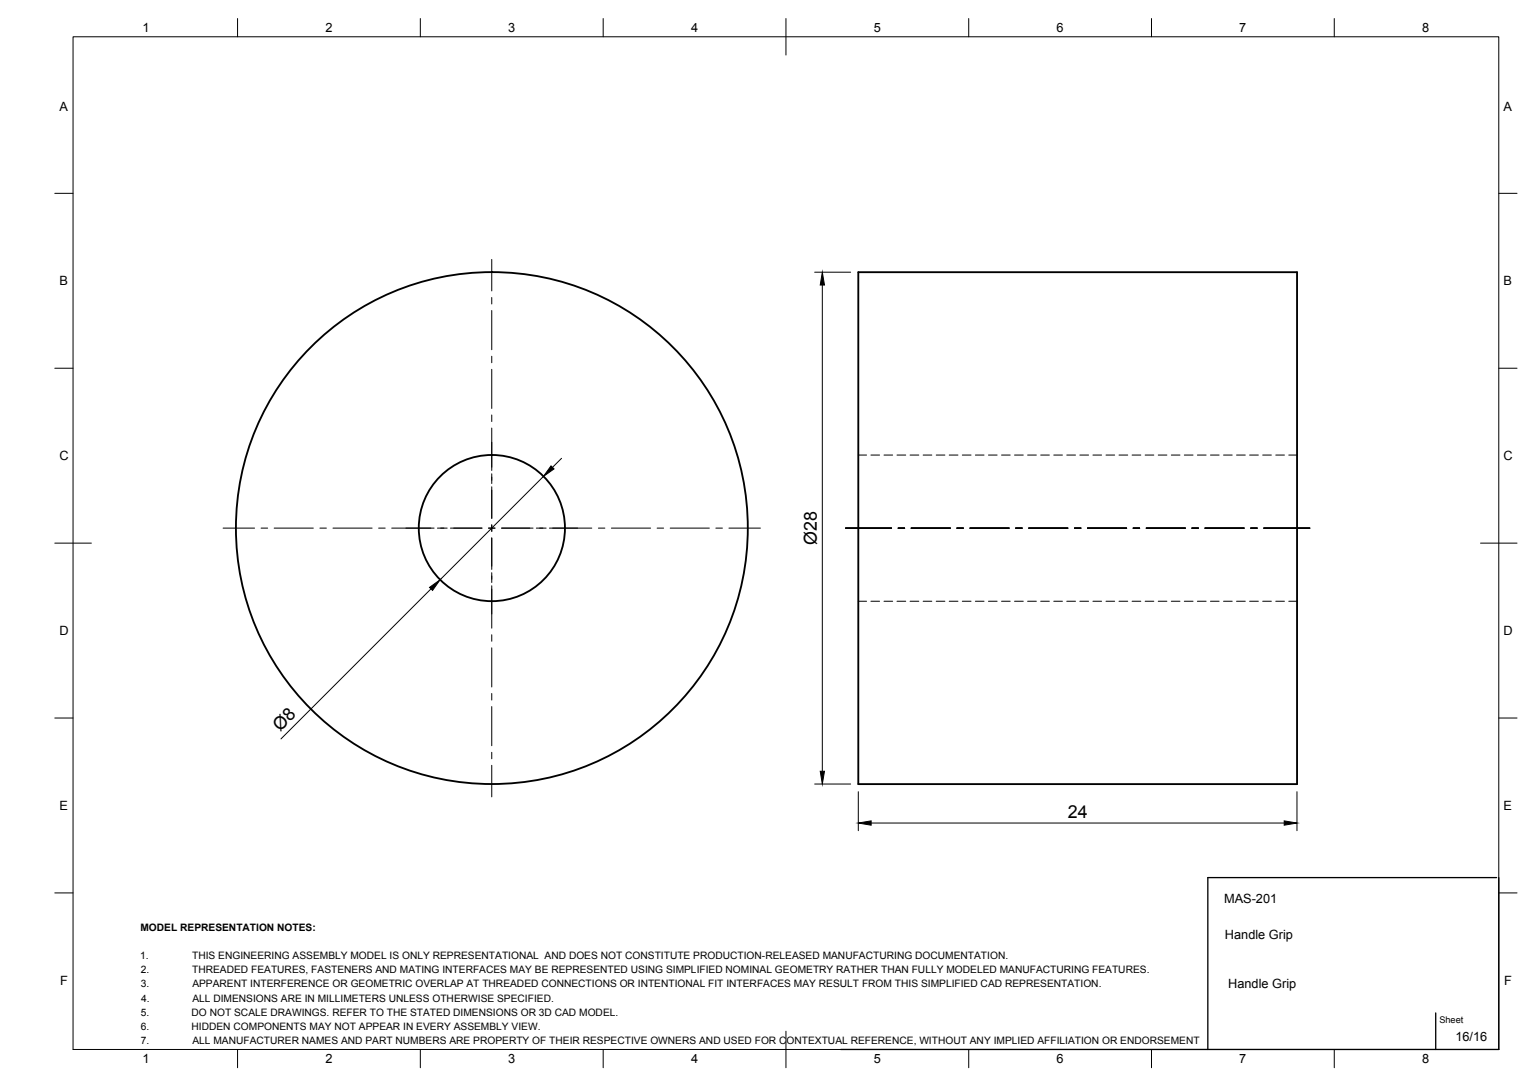
ISO-10303-21;
HEADER;
/* Generated by software containing ST-Developer
 * from STEP Tools, Inc. (www.steptools.com) 
 */

FILE_DESCRIPTION(
/* description */ ('Independent manual two-gate roller-track escapement for nominal30mm d
iameter20mm wide feed rollers. Opposed gates are driven by native capt
ured pin-slot loops with positive curved-slot travel stops at\X\B116de
g. Repeated gate/pin/washer/clip instances, adapted native common bear
ing families, full retaining lips and rotating polymer grip. External 
workpieces, gravity feeder/incline and mount anchors outside assembly.
 No powered-feed compatibility, impact, capacity, safety, force, wear 
or life rating.'),
/* implementation_level */ '2;1');

FILE_NAME(
/* name */ 'Handle grip.step',
/* time_stamp */ '2026-11-08T18:43:23-08:00',
/* author */ (''),
/* organization */ (''),
/* preprocessor_version */ 'ST-DEVELOPER v20.2',
/* originating_system */ 'Autodesk Translation Framework v15.17.0.0',
/* authorisation */ '');

FILE_SCHEMA (('AUTOMOTIVE_DESIGN { 1 0 10303 214 3 1 1 }'));
ENDSEC;

DATA;
#10=MECHANICAL_DESIGN_GEOMETRIC_PRESENTATION_REPRESENTATION('',(#471),#19863);
#433=SHAPE_REPRESENTATION_RELATIONSHIP('SRR','None',#19951,#452);
#452=ADVANCED_BREP_SHAPE_REPRESENTATION('',(#490),#19860);
#471=STYLED_ITEM('',(#20042),#490);
#490=MANIFOLD_SOLID_BREP('Body1',#6440);
#874=LINE('',#16034,#1339);
#875=LINE('',#16040,#1340);
#1339=VECTOR('',#8406,4.);
#1340=VECTOR('',#8413,12.);
#1566=CYLINDRICAL_SURFACE('',#7068,4.);
#1567=CYLINDRICAL_SURFACE('',#7071,14.);
#1680=FACE_BOUND('',#2391,.T.);
#1681=FACE_BOUND('',#2393,.T.);
#1966=FACE_OUTER_BOUND('',#2388,.T.);
#1967=FACE_OUTER_BOUND('',#2389,.T.);
#1968=FACE_OUTER_BOUND('',#2390,.T.);
#1969=FACE_OUTER_BOUND('',#2392,.T.);
#2388=EDGE_LOOP('',(#5505,#5506,#5507,#5508));
#2389=EDGE_LOOP('',(#5509,#5510,#5511,#5512));
#2390=EDGE_LOOP('',(#5513));
#2391=EDGE_LOOP('',(#5514));
#2392=EDGE_LOOP('',(#5515));
#2393=EDGE_LOOP('',(#5516));
#2598=CIRCLE('',#7069,4.);
#2599=CIRCLE('',#7070,4.);
#2600=CIRCLE('',#7072,14.);
#2601=CIRCLE('',#7073,14.);
#3080=VERTEX_POINT('',#16031);
#3081=VERTEX_POINT('',#16033);
#3082=VERTEX_POINT('',#16037);
#3083=VERTEX_POINT('',#16039);
#3911=EDGE_CURVE('',#3080,#3080,#2598,.T.);
#3912=EDGE_CURVE('',#3080,#3081,#874,.T.);
#3913=EDGE_CURVE('',#3081,#3081,#2599,.T.);
#3914=EDGE_CURVE('',#3082,#3082,#2600,.F.);
#3915=EDGE_CURVE('',#3082,#3083,#875,.T.);
#3916=EDGE_CURVE('',#3083,#3083,#2601,.F.);
#5505=ORIENTED_EDGE('',*,*,#3911,.F.);
#5506=ORIENTED_EDGE('',*,*,#3912,.T.);
#5507=ORIENTED_EDGE('',*,*,#3913,.T.);
#5508=ORIENTED_EDGE('',*,*,#3912,.F.);
#5509=ORIENTED_EDGE('',*,*,#3914,.F.);
#5510=ORIENTED_EDGE('',*,*,#3915,.T.);
#5511=ORIENTED_EDGE('',*,*,#3916,.T.);
#5512=ORIENTED_EDGE('',*,*,#3915,.F.);
#5513=ORIENTED_EDGE('',*,*,#3914,.T.);
#5514=ORIENTED_EDGE('',*,*,#3911,.T.);
#5515=ORIENTED_EDGE('',*,*,#3916,.F.);
#5516=ORIENTED_EDGE('',*,*,#3913,.F.);
#6043=PLANE('',#7074);
#6044=PLANE('',#7075);
#6345=ADVANCED_FACE('',(#1966),#1566,.F.);
#6346=ADVANCED_FACE('',(#1967),#1567,.T.);
#6347=ADVANCED_FACE('',(#1968,#1680),#6043,.T.);
#6348=ADVANCED_FACE('',(#1969,#1681),#6044,.F.);
#6440=CLOSED_SHELL('',(#6345,#6346,#6347,#6348));
#7067=AXIS2_PLACEMENT_3D('',#16029,#8400,#8401);
#7068=AXIS2_PLACEMENT_3D('',#16030,#8402,#8403);
#7069=AXIS2_PLACEMENT_3D('',#16032,#8404,#8405);
#7070=AXIS2_PLACEMENT_3D('',#16035,#8407,#8408);
#7071=AXIS2_PLACEMENT_3D('',#16036,#8409,#8410);
#7072=AXIS2_PLACEMENT_3D('',#16038,#8411,#8412);
#7073=AXIS2_PLACEMENT_3D('',#16041,#8414,#8415);
#7074=AXIS2_PLACEMENT_3D('',#16042,#8416,#8417);
#7075=AXIS2_PLACEMENT_3D('',#16043,#8418,#8419);
#8400=DIRECTION('axis',(0.,0.,1.));
#8401=DIRECTION('refdir',(1.,0.,0.));
#8402=DIRECTION('center_axis',(0.,0.,1.));
#8403=DIRECTION('ref_axis',(1.,0.,0.));
#8404=DIRECTION('center_axis',(0.,0.,-1.));
#8405=DIRECTION('ref_axis',(1.,0.,0.));
#8406=DIRECTION('',(0.,0.,-1.));
#8407=DIRECTION('center_axis',(0.,0.,-1.));
#8408=DIRECTION('ref_axis',(1.,0.,0.));
#8409=DIRECTION('center_axis',(0.,0.,1.));
#8410=DIRECTION('ref_axis',(1.,0.,0.));
#8411=DIRECTION('center_axis',(0.,0.,-1.));
#8412=DIRECTION('ref_axis',(1.,0.,0.));
#8413=DIRECTION('',(0.,0.,-1.));
#8414=DIRECTION('center_axis',(0.,0.,-1.));
#8415=DIRECTION('ref_axis',(1.,0.,0.));
#8416=DIRECTION('center_axis',(0.,0.,1.));
#8417=DIRECTION('ref_axis',(1.,0.,0.));
#8418=DIRECTION('center_axis',(0.,0.,1.));
#8419=DIRECTION('ref_axis',(1.,0.,0.));
#16029=CARTESIAN_POINT('',(0.,0.,0.));
#16030=CARTESIAN_POINT('Origin',(0.,0.,0.));
#16031=CARTESIAN_POINT('',(-4.,-4.89858719658941E-16,24.));
#16032=CARTESIAN_POINT('Origin',(0.,0.,24.));
#16033=CARTESIAN_POINT('',(-4.,-4.89858719658941E-16,0.));
#16034=CARTESIAN_POINT('',(-4.,-4.89858719658941E-16,0.));
#16035=CARTESIAN_POINT('Origin',(0.,0.,0.));
#16036=CARTESIAN_POINT('Origin',(0.,0.,0.));
#16037=CARTESIAN_POINT('',(-14.,1.71450551880629E-15,24.));
#16038=CARTESIAN_POINT('Origin',(0.,0.,24.));
#16039=CARTESIAN_POINT('',(-14.,1.71450551880629E-15,0.));
#16040=CARTESIAN_POINT('',(-14.,-1.71450551880629E-15,0.));
#16041=CARTESIAN_POINT('Origin',(0.,0.,0.));
#16042=CARTESIAN_POINT('Origin',(0.,0.,24.));
#16043=CARTESIAN_POINT('Origin',(0.,0.,0.));
#19839=UNCERTAINTY_MEASURE_WITH_UNIT(LENGTH_MEASURE(0.01),#19864,
'DISTANCE_ACCURACY_VALUE',
'Maximum model space distance between geometric entities at asserted c
onnectivities');
#19842=UNCERTAINTY_MEASURE_WITH_UNIT(LENGTH_MEASURE(0.01),#19864,
'DISTANCE_ACCURACY_VALUE',
'Maximum model space distance between geometric entities at asserted c
onnectivities');
#19860=(
GEOMETRIC_REPRESENTATION_CONTEXT(3)
GLOBAL_UNCERTAINTY_ASSIGNED_CONTEXT((#19839))
GLOBAL_UNIT_ASSIGNED_CONTEXT((#19864,#19866,#19867))
REPRESENTATION_CONTEXT('','3D')
);
#19863=(
GEOMETRIC_REPRESENTATION_CONTEXT(3)
GLOBAL_UNCERTAINTY_ASSIGNED_CONTEXT((#19842))
GLOBAL_UNIT_ASSIGNED_CONTEXT((#19864,#19866,#19867))
REPRESENTATION_CONTEXT('','3D')
);
#19864=(
LENGTH_UNIT()
NAMED_UNIT(*)
SI_UNIT(.MILLI.,.METRE.)
);
#19866=(
NAMED_UNIT(*)
PLANE_ANGLE_UNIT()
SI_UNIT($,.RADIAN.)
);
#19867=(
NAMED_UNIT(*)
SI_UNIT($,.STERADIAN.)
SOLID_ANGLE_UNIT()
);
#19885=SHAPE_DEFINITION_REPRESENTATION(#19905,#19951);
#19905=PRODUCT_DEFINITION_SHAPE('',$,#19972);
#19951=SHAPE_REPRESENTATION('',(#7067),#19860);
#19954=PRODUCT_DEFINITION_CONTEXT('part definition',#20016,'design');
#19972=PRODUCT_DEFINITION('Handle Grip','Handle grip',#19992,#19954);
#19992=PRODUCT_DEFINITION_FORMATION('',$,#20035);
#20016=APPLICATION_CONTEXT(
'Core Data for Automotive Mechanical Design Process');
#20017=PRODUCT_CONTEXT('part definition',#20016,'mechanical');
#20035=PRODUCT('Handle Grip','Handle grip',$,(#20017));
#20042=PRESENTATION_STYLE_ASSIGNMENT((#20049));
#20049=SURFACE_STYLE_USAGE(.BOTH.,#20056);
#20056=SURFACE_SIDE_STYLE('',(#20063));
#20063=SURFACE_STYLE_FILL_AREA(#20070);
#20070=FILL_AREA_STYLE('Gray',(#20077));
#20077=FILL_AREA_STYLE_COLOUR('Gray',#20084);
#20084=COLOUR_RGB('Gray',0.407843137254902,0.447058823529412,0.498039215686275);
ENDSEC;
END-ISO-10303-21;
